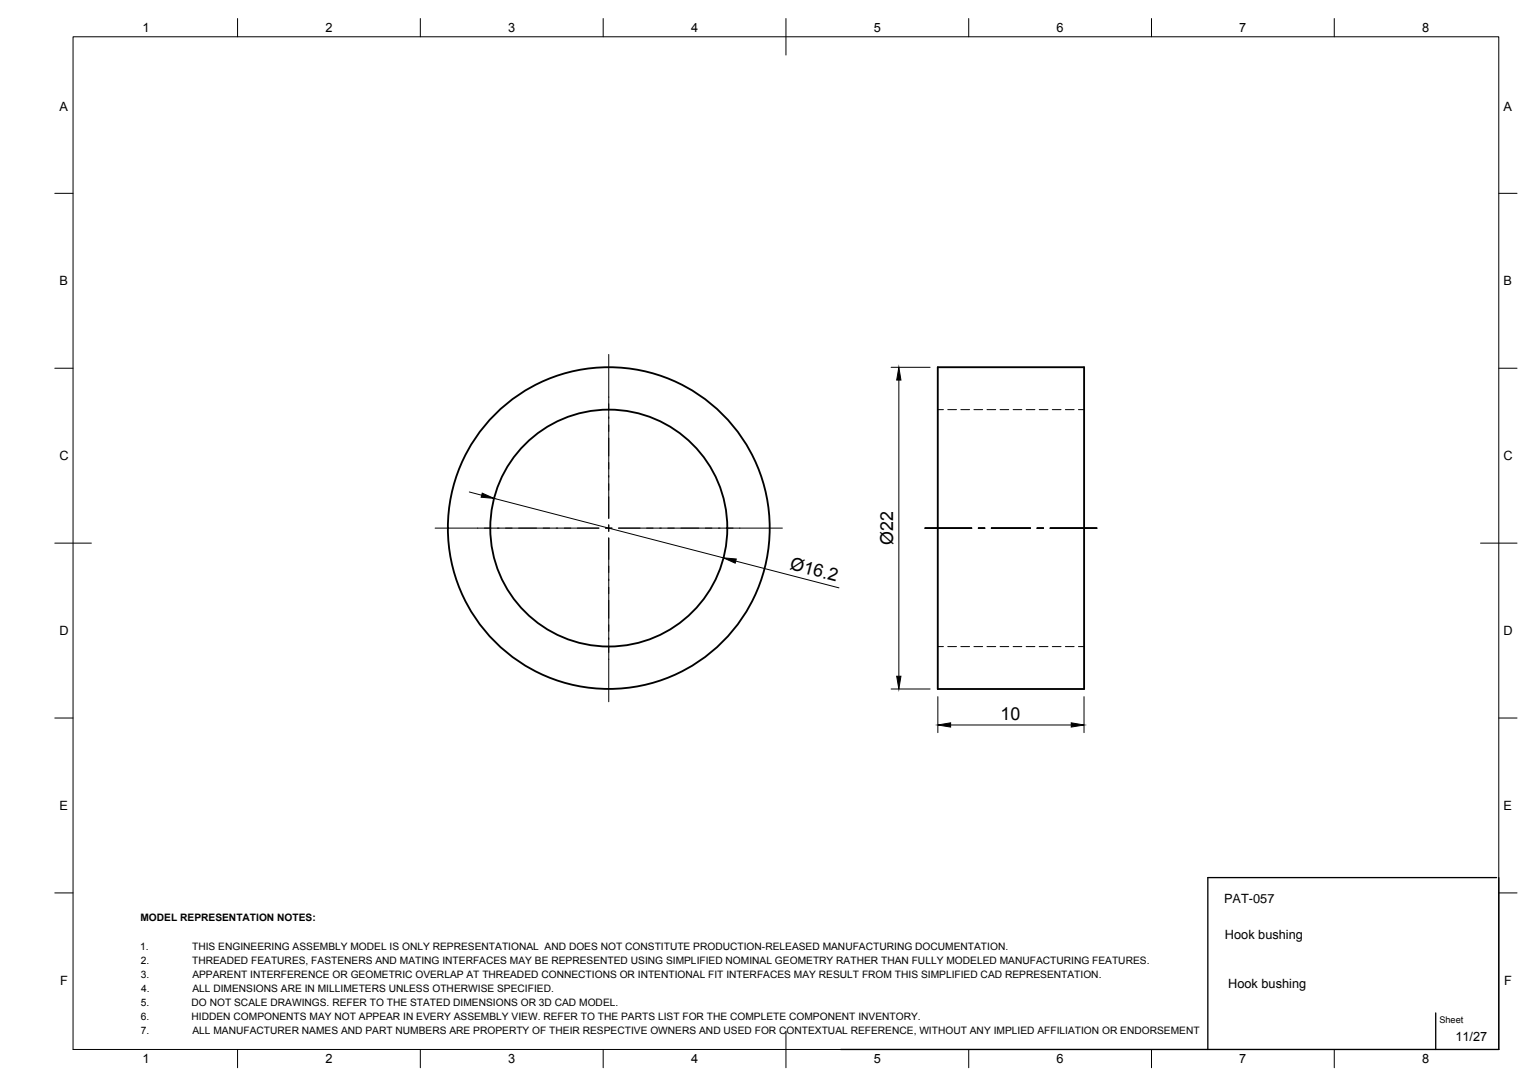
ISO-10303-21;
HEADER;
/* Generated by software containing ST-Developer
 * from STEP Tools, Inc. (www.steptools.com) 
 */

FILE_DESCRIPTION(
/* description */ ('Bearing-mounted hook block'),
/* implementation_level */ '2;1');

FILE_NAME(
/* name */ 'Hook bushing.step',
/* time_stamp */ '2026-10-28T22:30:11-07:00',
/* author */ (''),
/* organization */ (''),
/* preprocessor_version */ 'ST-DEVELOPER v20.2',
/* originating_system */ 'Autodesk Translation Framework v15.17.0.0',
/* authorisation */ '');

FILE_SCHEMA (('AUTOMOTIVE_DESIGN { 1 0 10303 214 3 1 1 }'));
ENDSEC;

DATA;
#10=MECHANICAL_DESIGN_GEOMETRIC_PRESENTATION_REPRESENTATION('',(#329),#7609);
#281=SHAPE_REPRESENTATION_RELATIONSHIP('SRR','None',#7728,#305);
#305=ADVANCED_BREP_SHAPE_REPRESENTATION('',(#361),#7588);
#329=STYLED_ITEM('',(#7917),#361);
#361=MANIFOLD_SOLID_BREP('Body1',#3925);
#449=LINE('',#6334,#679);
#450=LINE('',#6340,#680);
#679=VECTOR('',#5066,0.81);
#680=VECTOR('',#5073,1.1);
#869=CYLINDRICAL_SURFACE('',#4339,0.81);
#870=CYLINDRICAL_SURFACE('',#4342,1.1);
#949=FACE_BOUND('',#1321,.T.);
#950=FACE_BOUND('',#1323,.T.);
#1054=FACE_OUTER_BOUND('',#1318,.T.);
#1055=FACE_OUTER_BOUND('',#1319,.T.);
#1056=FACE_OUTER_BOUND('',#1320,.T.);
#1057=FACE_OUTER_BOUND('',#1322,.T.);
#1318=EDGE_LOOP('',(#2836,#2837,#2838,#2839));
#1319=EDGE_LOOP('',(#2840,#2841,#2842,#2843));
#1320=EDGE_LOOP('',(#2844));
#1321=EDGE_LOOP('',(#2845));
#1322=EDGE_LOOP('',(#2846));
#1323=EDGE_LOOP('',(#2847));
#1611=CIRCLE('',#4340,0.81);
#1612=CIRCLE('',#4341,0.81);
#1613=CIRCLE('',#4343,1.1);
#1614=CIRCLE('',#4344,1.1);
#1860=VERTEX_POINT('',#6331);
#1861=VERTEX_POINT('',#6333);
#1862=VERTEX_POINT('',#6337);
#1863=VERTEX_POINT('',#6339);
#2228=EDGE_CURVE('',#1860,#1860,#1611,.T.);
#2229=EDGE_CURVE('',#1860,#1861,#449,.T.);
#2230=EDGE_CURVE('',#1861,#1861,#1612,.T.);
#2231=EDGE_CURVE('',#1862,#1862,#1613,.T.);
#2232=EDGE_CURVE('',#1862,#1863,#450,.T.);
#2233=EDGE_CURVE('',#1863,#1863,#1614,.T.);
#2836=ORIENTED_EDGE('',*,*,#2228,.F.);
#2837=ORIENTED_EDGE('',*,*,#2229,.T.);
#2838=ORIENTED_EDGE('',*,*,#2230,.T.);
#2839=ORIENTED_EDGE('',*,*,#2229,.F.);
#2840=ORIENTED_EDGE('',*,*,#2231,.F.);
#2841=ORIENTED_EDGE('',*,*,#2232,.T.);
#2842=ORIENTED_EDGE('',*,*,#2233,.T.);
#2843=ORIENTED_EDGE('',*,*,#2232,.F.);
#2844=ORIENTED_EDGE('',*,*,#2231,.T.);
#2845=ORIENTED_EDGE('',*,*,#2228,.T.);
#2846=ORIENTED_EDGE('',*,*,#2233,.F.);
#2847=ORIENTED_EDGE('',*,*,#2230,.F.);
#3588=PLANE('',#4345);
#3589=PLANE('',#4346);
#3736=ADVANCED_FACE('',(#1054),#869,.F.);
#3737=ADVANCED_FACE('',(#1055),#870,.T.);
#3738=ADVANCED_FACE('',(#1056,#949),#3588,.T.);
#3739=ADVANCED_FACE('',(#1057,#950),#3589,.F.);
#3925=CLOSED_SHELL('',(#3736,#3737,#3738,#3739));
#4338=AXIS2_PLACEMENT_3D('',#6329,#5060,#5061);
#4339=AXIS2_PLACEMENT_3D('',#6330,#5062,#5063);
#4340=AXIS2_PLACEMENT_3D('',#6332,#5064,#5065);
#4341=AXIS2_PLACEMENT_3D('',#6335,#5067,#5068);
#4342=AXIS2_PLACEMENT_3D('',#6336,#5069,#5070);
#4343=AXIS2_PLACEMENT_3D('',#6338,#5071,#5072);
#4344=AXIS2_PLACEMENT_3D('',#6341,#5074,#5075);
#4345=AXIS2_PLACEMENT_3D('',#6342,#5076,#5077);
#4346=AXIS2_PLACEMENT_3D('',#6343,#5078,#5079);
#5060=DIRECTION('axis',(0.,0.,1.));
#5061=DIRECTION('refdir',(1.,0.,0.));
#5062=DIRECTION('center_axis',(0.,0.,1.));
#5063=DIRECTION('ref_axis',(1.,0.,0.));
#5064=DIRECTION('center_axis',(0.,0.,-1.));
#5065=DIRECTION('ref_axis',(1.,0.,0.));
#5066=DIRECTION('',(0.,0.,-1.));
#5067=DIRECTION('center_axis',(0.,0.,-1.));
#5068=DIRECTION('ref_axis',(1.,0.,0.));
#5069=DIRECTION('center_axis',(0.,0.,1.));
#5070=DIRECTION('ref_axis',(1.,0.,0.));
#5071=DIRECTION('center_axis',(0.,0.,1.));
#5072=DIRECTION('ref_axis',(1.,0.,0.));
#5073=DIRECTION('',(0.,0.,-1.));
#5074=DIRECTION('center_axis',(0.,0.,1.));
#5075=DIRECTION('ref_axis',(1.,0.,0.));
#5076=DIRECTION('center_axis',(0.,0.,1.));
#5077=DIRECTION('ref_axis',(1.,0.,0.));
#5078=DIRECTION('center_axis',(0.,0.,1.));
#5079=DIRECTION('ref_axis',(1.,0.,0.));
#6329=CARTESIAN_POINT('',(0.,0.,0.));
#6330=CARTESIAN_POINT('Origin',(0.,0.,4.5));
#6331=CARTESIAN_POINT('',(-0.81,-9.91963907309356E-17,5.5));
#6332=CARTESIAN_POINT('Origin',(0.,0.,5.5));
#6333=CARTESIAN_POINT('',(-0.81,-9.91963907309356E-17,4.5));
#6334=CARTESIAN_POINT('',(-0.81,-9.91963907309356E-17,4.5));
#6335=CARTESIAN_POINT('Origin',(0.,0.,4.5));
#6336=CARTESIAN_POINT('Origin',(0.,0.,4.5));
#6337=CARTESIAN_POINT('',(-1.1,-1.34711147906209E-16,5.5));
#6338=CARTESIAN_POINT('Origin',(0.,0.,5.5));
#6339=CARTESIAN_POINT('',(-1.1,-1.34711147906209E-16,4.5));
#6340=CARTESIAN_POINT('',(-1.1,-1.34711147906209E-16,4.5));
#6341=CARTESIAN_POINT('Origin',(0.,0.,4.5));
#6342=CARTESIAN_POINT('Origin',(0.,0.,5.5));
#6343=CARTESIAN_POINT('Origin',(0.,0.,4.5));
#7558=UNCERTAINTY_MEASURE_WITH_UNIT(LENGTH_MEASURE(0.001),#7610,
'DISTANCE_ACCURACY_VALUE',
'Maximum model space distance between geometric entities at asserted c
onnectivities');
#7579=UNCERTAINTY_MEASURE_WITH_UNIT(LENGTH_MEASURE(0.001),#7610,
'DISTANCE_ACCURACY_VALUE',
'Maximum model space distance between geometric entities at asserted c
onnectivities');
#7588=(
GEOMETRIC_REPRESENTATION_CONTEXT(3)
GLOBAL_UNCERTAINTY_ASSIGNED_CONTEXT((#7558))
GLOBAL_UNIT_ASSIGNED_CONTEXT((#7610,#7612,#7613))
REPRESENTATION_CONTEXT('','3D')
);
#7609=(
GEOMETRIC_REPRESENTATION_CONTEXT(3)
GLOBAL_UNCERTAINTY_ASSIGNED_CONTEXT((#7579))
GLOBAL_UNIT_ASSIGNED_CONTEXT((#7610,#7612,#7613))
REPRESENTATION_CONTEXT('','3D')
);
#7610=(
LENGTH_UNIT()
NAMED_UNIT(*)
SI_UNIT(.CENTI.,.METRE.)
);
#7612=(
NAMED_UNIT(*)
PLANE_ANGLE_UNIT()
SI_UNIT($,.RADIAN.)
);
#7613=(
NAMED_UNIT(*)
SI_UNIT($,.STERADIAN.)
SOLID_ANGLE_UNIT()
);
#7622=SHAPE_DEFINITION_REPRESENTATION(#7651,#7728);
#7651=PRODUCT_DEFINITION_SHAPE('',$,#7758);
#7728=SHAPE_REPRESENTATION('',(#4338),#7588);
#7749=PRODUCT_DEFINITION_CONTEXT('part definition',#7838,'design');
#7758=PRODUCT_DEFINITION('Hook bushing','Hook bushing',#7787,#7749);
#7787=PRODUCT_DEFINITION_FORMATION('',$,#7848);
#7838=APPLICATION_CONTEXT(
'Core Data for Automotive Mechanical Design Process');
#7839=PRODUCT_CONTEXT('part definition',#7838,'mechanical');
#7848=PRODUCT('Hook bushing','Hook bushing','Hook bushing',(#7839));
#7911=COLOUR_RGB('Light Blue',0.38,0.62,0.78);
#7912=FILL_AREA_STYLE_COLOUR('',#7911);
#7913=FILL_AREA_STYLE('',(#7912));
#7914=SURFACE_STYLE_FILL_AREA(#7913);
#7915=SURFACE_SIDE_STYLE('',(#7914));
#7916=SURFACE_STYLE_USAGE(.BOTH.,#7915);
#7917=PRESENTATION_STYLE_ASSIGNMENT((#7916));
ENDSEC;
END-ISO-10303-21;
